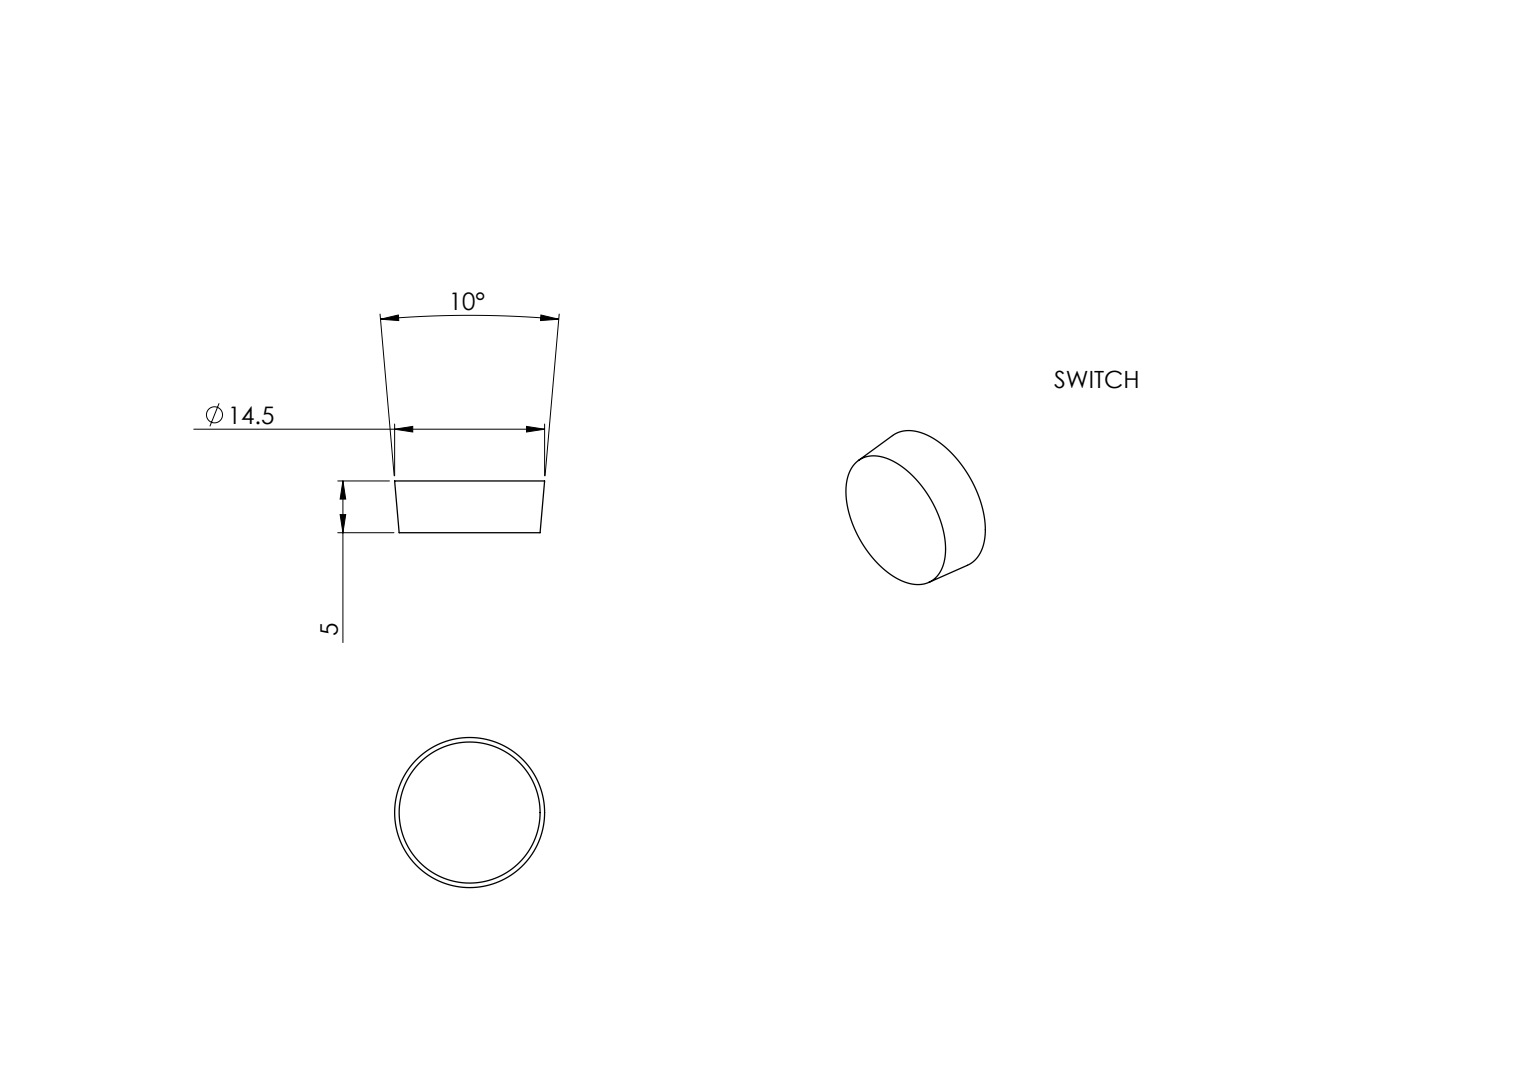
ISO-10303-21;
HEADER;
FILE_DESCRIPTION (('STEP AP214'),
    '1' );
FILE_NAME ('switch^MAS-192.step',
    '2026-10-24T04:45:50',
    ( '' ),
    ( '' ),
    'SwSTEP 2.0',
    'SolidWorks 2026',
    '' );
FILE_SCHEMA (( 'AUTOMOTIVE_DESIGN' ));
ENDSEC;

DATA;
#44=AXIS2_PLACEMENT_3D ( 'NONE', #1214, #1923, #390 ) ;
#47=AXIS2_PLACEMENT_3D ( 'NONE', #2108, #1339, #2131 ) ;
#101=CONICAL_SURFACE ( 'NONE', #2881, 7.250000000000000000, 0.08726646259971666819 ) ;
#109=( GEOMETRIC_REPRESENTATION_CONTEXT ( 3 ) GLOBAL_UNCERTAINTY_ASSIGNED_CONTEXT ( ( #1070 ) ) GLOBAL_UNIT_ASSIGNED_CONTEXT ( ( #2231, #2739, #2029 ) ) REPRESENTATION_CONTEXT ( 'NONE', 'WORKASPACE' ) );
#129=SURFACE_STYLE_FILL_AREA ( #3049 ) ;
#188=ORIENTED_EDGE ( 'NONE', *, *, #783, .T. ) ;
#202=CIRCLE ( 'NONE', #44, 6.812556682370379590 ) ;
#240=PRODUCT_DEFINITION_CONTEXT ( 'detailed design', #1502, 'design' ) ;
#255=ORIENTED_EDGE ( 'NONE', *, *, #1651, .T. ) ;
#276=CARTESIAN_POINT ( 'NONE',  ( 7.250000000000000000, 25.00000000000000000, 47.00000000000000000 ) ) ;
#317=CIRCLE ( 'NONE', #47, 7.250000000000000000 ) ;
#329=MECHANICAL_DESIGN_GEOMETRIC_PRESENTATION_REPRESENTATION('',(#1259),#109);
#342=DIRECTION ( 'NONE',  ( 1.000000000000000000, 0.000000000000000000, 0.000000000000000000 ) ) ;
#390=DIRECTION ( 'NONE',  ( 1.000000000000000000, 0.000000000000000000, 0.000000000000000000 ) ) ;
#489=VERTEX_POINT ( 'NONE', #1686 ) ;
#503=EDGE_CURVE ( 'NONE', #2959, #3196, #202, .T. ) ;
#516=ADVANCED_BREP_SHAPE_REPRESENTATION ( '', ( #3171, #3111 ), #2779 ) ;
#518=ADVANCED_FACE ( 'NONE', ( #2751 ), #3260, .T. ) ;
#560=DIRECTION ( 'NONE',  ( 0.08715574274765836016, 0.000000000000000000, -0.9961946980917455452 ) ) ;
#586=AXIS2_PLACEMENT_3D ( 'NONE', #2582, #2295, #1015 ) ;
#602=EDGE_LOOP ( 'NONE', ( #1760, #2359 ) ) ;
#613=ORIENTED_EDGE ( 'NONE', *, *, #2891, .T. ) ;
#615=UNCERTAINTY_MEASURE_WITH_UNIT (LENGTH_MEASURE( 1.000000000000000082E-05 ), #1164, 'distance_accuracy_value', 'NONE');
#628=ORIENTED_EDGE ( 'NONE', *, *, #2891, .F. ) ;
#638=CARTESIAN_POINT ( 'NONE',  ( 0.000000000000000000, 25.00000000000000000, 52.00000000000000000 ) ) ;
#675=CARTESIAN_POINT ( 'NONE',  ( -6.812556682370379590, 25.00000000000000000, 52.00000000000000000 ) ) ;
#693=AXIS2_PLACEMENT_3D ( 'NONE', #3363, #1018, #2650 ) ;
#738=APPLICATION_CONTEXT ( 'automotive_design' ) ;
#769=COLOUR_RGB ( '',0.8941176470588234615, 0.8941176470588234615, 0.8941176470588234615 ) ;
#783=EDGE_CURVE ( 'NONE', #3196, #489, #2960, .T. ) ;
#825=EDGE_CURVE ( 'NONE', #3196, #2959, #3040, .T. ) ;
#840=DIRECTION ( 'NONE',  ( 0.000000000000000000, 0.000000000000000000, 1.000000000000000000 ) ) ;
#852=ORIENTED_EDGE ( 'NONE', *, *, #503, .F. ) ;
#860=CONICAL_SURFACE ( 'NONE', #693, 7.250000000000000000, 0.08726646259971666819 ) ;
#911=( LENGTH_UNIT ( ) NAMED_UNIT ( * ) SI_UNIT ( .MILLI., .METRE. ) );
#936=SHAPE_REPRESENTATION ( 'switch^MAS-192', ( #3111 ), #2779 ) ;
#973=AXIS2_PLACEMENT_3D ( 'NONE', #1897, #840, #2668 ) ;
#988=PRODUCT_DEFINITION_FORMATION_WITH_SPECIFIED_SOURCE ( 'ANY', '', #1577, .NOT_KNOWN. ) ;
#1015=DIRECTION ( 'NONE',  ( 1.000000000000000000, 0.000000000000000000, -0.000000000000000000 ) ) ;
#1018=DIRECTION ( 'NONE',  ( -0.000000000000000000, -0.000000000000000000, -1.000000000000000000 ) ) ;
#1070=UNCERTAINTY_MEASURE_WITH_UNIT (LENGTH_MEASURE( 1.000000000000000082E-05 ), #2231, 'distance_accuracy_value', 'NONE');
#1085=AXIS2_PLACEMENT_3D ( 'NONE', #1615, #3162, #1636 ) ;
#1164=( LENGTH_UNIT ( ) NAMED_UNIT ( * ) SI_UNIT ( .MILLI., .METRE. ) );
#1189=( NAMED_UNIT ( * ) PLANE_ANGLE_UNIT ( ) SI_UNIT ( $, .RADIAN. ) );
#1214=CARTESIAN_POINT ( 'NONE',  ( 0.000000000000000000, 25.00000000000000000, 52.00000000000000000 ) ) ;
#1243=ADVANCED_FACE ( 'NONE', ( #2970 ), #101, .T. ) ;
#1259=STYLED_ITEM('',(#3415),#3171);
#1283=LINE ( 'NONE', #276, #2395 ) ;
#1297=VERTEX_POINT ( 'NONE', #1740 ) ;
#1312=DIRECTION ( 'NONE',  ( -0.08715574274765836016, -1.067350013832299517E-17, -0.9961946980917455452 ) ) ;
#1313=STYLED_ITEM ( 'NONE', ( #2530 ), #516 ) ;
#1339=DIRECTION ( 'NONE',  ( 0.000000000000000000, 0.000000000000000000, 1.000000000000000000 ) ) ;
#1404=AXIS2_PLACEMENT_3D ( 'NONE', #638, #1429, #1972 ) ;
#1419=DIRECTION ( 'NONE',  ( -0.000000000000000000, -0.000000000000000000, -1.000000000000000000 ) ) ;
#1429=DIRECTION ( 'NONE',  ( 0.000000000000000000, 0.000000000000000000, 1.000000000000000000 ) ) ;
#1502=APPLICATION_CONTEXT ( 'automotive_design' ) ;
#1544=SHAPE_REPRESENTATION_RELATIONSHIP ( 'NONE' , 'NONE' ,  #936, #516 ) ;
#1577=PRODUCT ( 'switch^MAS-192', 'switch^MAS-192', '', ( #3242 ) ) ;
#1615=CARTESIAN_POINT ( 'NONE',  ( 0.000000000000000000, 25.00000000000000000, 47.00000000000000000 ) ) ;
#1636=DIRECTION ( 'NONE',  ( 1.000000000000000000, 0.000000000000000000, 0.000000000000000000 ) ) ;
#1651=EDGE_CURVE ( 'NONE', #1297, #489, #2449, .T. ) ;
#1686=CARTESIAN_POINT ( 'NONE',  ( -7.250000000000000000, 25.00000000000000000, 47.00000000000000000 ) ) ;
#1740=CARTESIAN_POINT ( 'NONE',  ( 7.250000000000000000, 25.00000000000000000, 47.00000000000000000 ) ) ;
#1760=ORIENTED_EDGE ( 'NONE', *, *, #503, .T. ) ;
#1777=ORIENTED_EDGE ( 'NONE', *, *, #825, .F. ) ;
#1783=FACE_OUTER_BOUND ( 'NONE', #2038, .T. ) ;
#1871=CARTESIAN_POINT ( 'NONE',  ( 0.000000000000000000, 0.000000000000000000, 0.000000000000000000 ) ) ;
#1897=CARTESIAN_POINT ( 'NONE',  ( 0.000000000000000000, 25.00000000000000000, 52.00000000000000000 ) ) ;
#1903=EDGE_LOOP ( 'NONE', ( #2092, #852, #613, #255 ) ) ;
#1923=DIRECTION ( 'NONE',  ( 0.000000000000000000, 0.000000000000000000, 1.000000000000000000 ) ) ;
#1971=SURFACE_SIDE_STYLE ('',( #129 ) ) ;
#1972=DIRECTION ( 'NONE',  ( 1.000000000000000000, 0.000000000000000000, -0.000000000000000000 ) ) ;
#2025=PRODUCT_DEFINITION ( 'UNKNOWN', '', #988, #240 ) ;
#2029=( NAMED_UNIT ( * ) SI_UNIT ( $, .STERADIAN. ) SOLID_ANGLE_UNIT ( ) );
#2038=EDGE_LOOP ( 'NONE', ( #1777, #188, #2145, #628 ) ) ;
#2071=ADVANCED_FACE ( 'NONE', ( #1783 ), #860, .T. ) ;
#2092=ORIENTED_EDGE ( 'NONE', *, *, #783, .F. ) ;
#2108=CARTESIAN_POINT ( 'NONE',  ( 0.000000000000000000, 25.00000000000000000, 47.00000000000000000 ) ) ;
#2131=DIRECTION ( 'NONE',  ( 1.000000000000000000, 0.000000000000000000, 0.000000000000000000 ) ) ;
#2137=CARTESIAN_POINT ( 'NONE',  ( 6.812556682370379590, 25.00000000000000000, 52.00000000000000000 ) ) ;
#2143=EDGE_CURVE ( 'NONE', #489, #1297, #317, .T. ) ;
#2145=ORIENTED_EDGE ( 'NONE', *, *, #2143, .T. ) ;
#2231=( LENGTH_UNIT ( ) NAMED_UNIT ( * ) SI_UNIT ( .MILLI., .METRE. ) );
#2293=UNCERTAINTY_MEASURE_WITH_UNIT (LENGTH_MEASURE( 1.000000000000000082E-05 ), #911, 'distance_accuracy_value', 'NONE');
#2295=DIRECTION ( 'NONE',  ( 0.000000000000000000, 0.000000000000000000, 1.000000000000000000 ) ) ;
#2311=FACE_OUTER_BOUND ( 'NONE', #2766, .T. ) ;
#2359=ORIENTED_EDGE ( 'NONE', *, *, #825, .T. ) ;
#2395=VECTOR ( 'NONE', #560, 1000.000000000000000 ) ;
#2425=CARTESIAN_POINT ( 'NONE',  ( -7.250000000000000000, 25.00000000000000000, 47.00000000000000000 ) ) ;
#2448=SHAPE_DEFINITION_REPRESENTATION ( #3352, #936 ) ;
#2449=CIRCLE ( 'NONE', #1085, 7.250000000000000000 ) ;
#2455=( GEOMETRIC_REPRESENTATION_CONTEXT ( 3 ) GLOBAL_UNCERTAINTY_ASSIGNED_CONTEXT ( ( #615 ) ) GLOBAL_UNIT_ASSIGNED_CONTEXT ( ( #1164, #2773, #2843 ) ) REPRESENTATION_CONTEXT ( 'NONE', 'WORKASPACE' ) );
#2458=ADVANCED_FACE ( 'NONE', ( #2311 ), #2856, .F. ) ;
#2507=MECHANICAL_DESIGN_GEOMETRIC_PRESENTATION_REPRESENTATION('',(#1313),#2455);
#2530=PRESENTATION_STYLE_ASSIGNMENT (( #2750 ) ) ;
#2582=CARTESIAN_POINT ( 'NONE',  ( 0.000000000000000000, 25.00000000000000000, 47.00000000000000000 ) ) ;
#2604=VECTOR ( 'NONE', #1312, 1000.000000000000000 ) ;
#2639=DIRECTION ( 'NONE',  ( 1.000000000000000000, 0.000000000000000000, 0.000000000000000000 ) ) ;
#2649=ORIENTED_EDGE ( 'NONE', *, *, #2143, .F. ) ;
#2650=DIRECTION ( 'NONE',  ( 1.000000000000000000, 0.000000000000000000, 0.000000000000000000 ) ) ;
#2668=DIRECTION ( 'NONE',  ( 1.000000000000000000, 0.000000000000000000, 0.000000000000000000 ) ) ;
#2708=CARTESIAN_POINT ( 'NONE',  ( 0.000000000000000000, 25.00000000000000000, 47.00000000000000000 ) ) ;
#2721=FILL_AREA_STYLE_COLOUR ( '', #769 ) ;
#2739=( NAMED_UNIT ( * ) PLANE_ANGLE_UNIT ( ) SI_UNIT ( $, .RADIAN. ) );
#2750=SURFACE_STYLE_USAGE ( .BOTH. , #1971 ) ;
#2751=FACE_OUTER_BOUND ( 'NONE', #602, .T. ) ;
#2766=EDGE_LOOP ( 'NONE', ( #3061, #2649 ) ) ;
#2773=( NAMED_UNIT ( * ) PLANE_ANGLE_UNIT ( ) SI_UNIT ( $, .RADIAN. ) );
#2779=( GEOMETRIC_REPRESENTATION_CONTEXT ( 3 ) GLOBAL_UNCERTAINTY_ASSIGNED_CONTEXT ( ( #2293 ) ) GLOBAL_UNIT_ASSIGNED_CONTEXT ( ( #911, #1189, #3014 ) ) REPRESENTATION_CONTEXT ( 'NONE', 'WORKASPACE' ) );
#2843=( NAMED_UNIT ( * ) SI_UNIT ( $, .STERADIAN. ) SOLID_ANGLE_UNIT ( ) );
#2856=PLANE ( 'NONE',  #586 ) ;
#2881=AXIS2_PLACEMENT_3D ( 'NONE', #2708, #1419, #342 ) ;
#2891=EDGE_CURVE ( 'NONE', #2959, #1297, #1283, .T. ) ;
#2923=CLOSED_SHELL ( 'NONE', ( #2071, #1243, #518, #2458 ) ) ;
#2959=VERTEX_POINT ( 'NONE', #2137 ) ;
#2960=LINE ( 'NONE', #2425, #2604 ) ;
#2970=FACE_OUTER_BOUND ( 'NONE', #1903, .T. ) ;
#3014=( NAMED_UNIT ( * ) SI_UNIT ( $, .STERADIAN. ) SOLID_ANGLE_UNIT ( ) );
#3040=CIRCLE ( 'NONE', #973, 6.812556682370379590 ) ;
#3049=FILL_AREA_STYLE ('',( #2721 ) ) ;
#3061=ORIENTED_EDGE ( 'NONE', *, *, #1651, .F. ) ;
#3111=AXIS2_PLACEMENT_3D ( 'NONE', #1871, #3207, #2639 ) ;
#3162=DIRECTION ( 'NONE',  ( 0.000000000000000000, 0.000000000000000000, 1.000000000000000000 ) ) ;
#3171=MANIFOLD_SOLID_BREP ( 'Boss-Extrude1', #2923 ) ;
#3196=VERTEX_POINT ( 'NONE', #675 ) ;
#3207=DIRECTION ( 'NONE',  ( 0.000000000000000000, 0.000000000000000000, 1.000000000000000000 ) ) ;
#3242=PRODUCT_CONTEXT ( 'NONE', #738, 'mechanical' ) ;
#3260=PLANE ( 'NONE',  #1404 ) ;
#3352=PRODUCT_DEFINITION_SHAPE ( 'NONE', 'NONE',  #2025 ) ;
#3363=CARTESIAN_POINT ( 'NONE',  ( 0.000000000000000000, 25.00000000000000000, 47.00000000000000000 ) ) ;
#3409=COLOUR_RGB('Grey',0.48,0.52,0.57);
#3410=FILL_AREA_STYLE_COLOUR('',#3409);
#3411=FILL_AREA_STYLE('',(#3410));
#3412=SURFACE_STYLE_FILL_AREA(#3411);
#3413=SURFACE_SIDE_STYLE('',(#3412));
#3414=SURFACE_STYLE_USAGE(.BOTH.,#3413);
#3415=PRESENTATION_STYLE_ASSIGNMENT((#3414));
ENDSEC;
END-ISO-10303-21;
